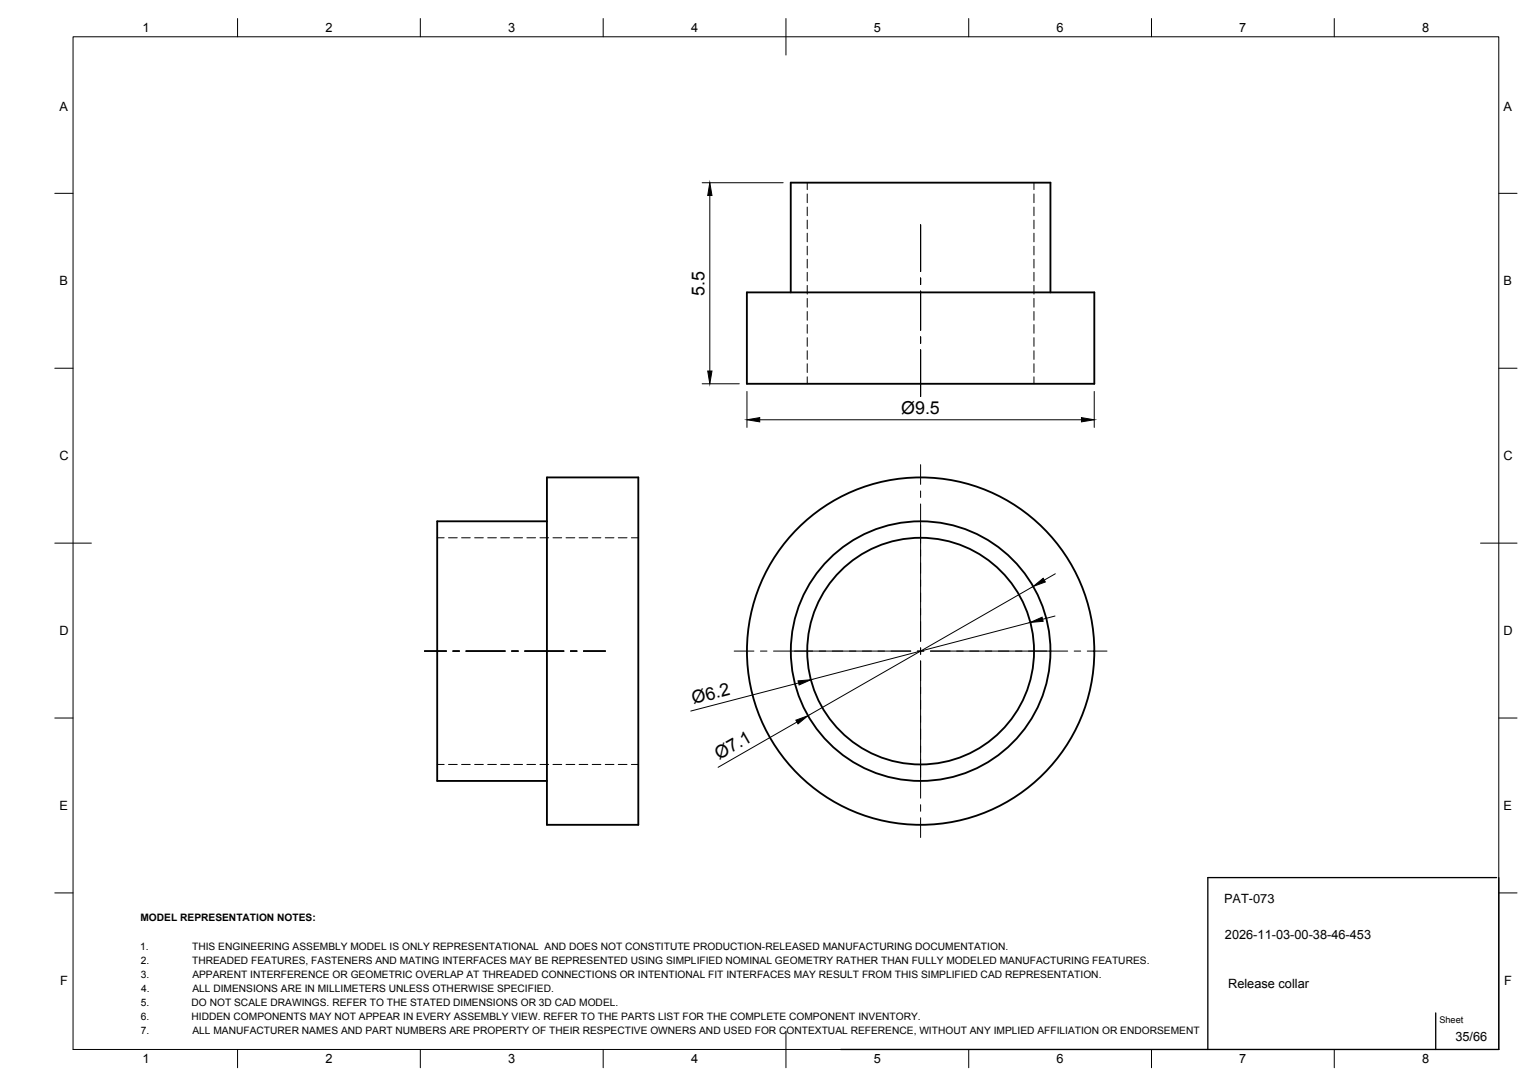
ISO-10303-21;
HEADER;
/* Generated by software containing ST-Developer
 * from STEP Tools, Inc. (www.steptools.com) 
 */

FILE_DESCRIPTION(
/* description */ ('Manual piston pump'),
/* implementation_level */ '2;1');

FILE_NAME(
/* name */ 'Release collar.step',
/* time_stamp */ '2026-11-02T16:54:23-08:00',
/* author */ (''),
/* organization */ (''),
/* preprocessor_version */ 'ST-DEVELOPER v20.2',
/* originating_system */ 'Autodesk Translation Framework v15.17.0.0',
/* authorisation */ '');

FILE_SCHEMA (('AUTOMOTIVE_DESIGN { 1 0 10303 214 3 1 1 }'));
ENDSEC;

DATA;
#10=MECHANICAL_DESIGN_GEOMETRIC_PRESENTATION_REPRESENTATION('',(#729),#19043);
#595=SHAPE_REPRESENTATION_RELATIONSHIP('SRR','None',#19343,#658);
#658=ADVANCED_BREP_SHAPE_REPRESENTATION('',(#799),#19010);
#729=STYLED_ITEM('',(#19661),#799);
#799=MANIFOLD_SOLID_BREP('Body1',#9515);
#990=FACE_BOUND('',#2393,.T.);
#991=FACE_BOUND('',#2396,.T.);
#992=FACE_BOUND('',#2399,.T.);
#1227=CYLINDRICAL_SURFACE('',#10992,0.475);
#1228=CYLINDRICAL_SURFACE('',#10996,0.355);
#1229=CYLINDRICAL_SURFACE('',#11000,0.31);
#1654=FACE_OUTER_BOUND('',#2392,.T.);
#1655=FACE_OUTER_BOUND('',#2394,.T.);
#1656=FACE_OUTER_BOUND('',#2395,.T.);
#1657=FACE_OUTER_BOUND('',#2397,.T.);
#1658=FACE_OUTER_BOUND('',#2398,.T.);
#1659=FACE_OUTER_BOUND('',#2400,.T.);
#2392=EDGE_LOOP('',(#7773));
#2393=EDGE_LOOP('',(#7774));
#2394=EDGE_LOOP('',(#7775,#7776,#7777,#7778));
#2395=EDGE_LOOP('',(#7779));
#2396=EDGE_LOOP('',(#7780));
#2397=EDGE_LOOP('',(#7781,#7782,#7783,#7784));
#2398=EDGE_LOOP('',(#7785));
#2399=EDGE_LOOP('',(#7786));
#2400=EDGE_LOOP('',(#7787,#7788,#7789,#7790));
#2998=CIRCLE('',#10990,0.475);
#2999=CIRCLE('',#10991,0.31);
#3000=CIRCLE('',#10993,0.475);
#3001=CIRCLE('',#10995,0.355);
#3002=CIRCLE('',#10997,0.355);
#3003=CIRCLE('',#10999,0.31);
#3517=LINE('',#17256,#4121);
#3518=LINE('',#17263,#4122);
#3519=LINE('',#17268,#4123);
#4121=VECTOR('',#13367,0.475);
#4122=VECTOR('',#13376,0.355);
#4123=VECTOR('',#13383,0.31);
#4860=VERTEX_POINT('',#17249);
#4861=VERTEX_POINT('',#17251);
#4862=VERTEX_POINT('',#17254);
#4863=VERTEX_POINT('',#17258);
#4864=VERTEX_POINT('',#17261);
#4865=VERTEX_POINT('',#17265);
#5873=EDGE_CURVE('',#4860,#4860,#2998,.T.);
#5874=EDGE_CURVE('',#4861,#4861,#2999,.T.);
#5875=EDGE_CURVE('',#4862,#4862,#3000,.T.);
#5876=EDGE_CURVE('',#4862,#4860,#3517,.T.);
#5877=EDGE_CURVE('',#4863,#4863,#3001,.T.);
#5878=EDGE_CURVE('',#4864,#4864,#3002,.T.);
#5879=EDGE_CURVE('',#4864,#4863,#3518,.T.);
#5880=EDGE_CURVE('',#4865,#4865,#3003,.T.);
#5881=EDGE_CURVE('',#4865,#4861,#3519,.T.);
#7773=ORIENTED_EDGE('',*,*,#5873,.F.);
#7774=ORIENTED_EDGE('',*,*,#5874,.T.);
#7775=ORIENTED_EDGE('',*,*,#5875,.F.);
#7776=ORIENTED_EDGE('',*,*,#5876,.T.);
#7777=ORIENTED_EDGE('',*,*,#5873,.T.);
#7778=ORIENTED_EDGE('',*,*,#5876,.F.);
#7779=ORIENTED_EDGE('',*,*,#5875,.T.);
#7780=ORIENTED_EDGE('',*,*,#5877,.F.);
#7781=ORIENTED_EDGE('',*,*,#5878,.F.);
#7782=ORIENTED_EDGE('',*,*,#5879,.T.);
#7783=ORIENTED_EDGE('',*,*,#5877,.T.);
#7784=ORIENTED_EDGE('',*,*,#5879,.F.);
#7785=ORIENTED_EDGE('',*,*,#5878,.T.);
#7786=ORIENTED_EDGE('',*,*,#5880,.F.);
#7787=ORIENTED_EDGE('',*,*,#5880,.T.);
#7788=ORIENTED_EDGE('',*,*,#5881,.T.);
#7789=ORIENTED_EDGE('',*,*,#5874,.F.);
#7790=ORIENTED_EDGE('',*,*,#5881,.F.);
#8764=PLANE('',#10989);
#8765=PLANE('',#10994);
#8766=PLANE('',#10998);
#9259=ADVANCED_FACE('',(#1654,#990),#8764,.T.);
#9260=ADVANCED_FACE('',(#1655),#1227,.T.);
#9261=ADVANCED_FACE('',(#1656,#991),#8765,.T.);
#9262=ADVANCED_FACE('',(#1657),#1228,.T.);
#9263=ADVANCED_FACE('',(#1658,#992),#8766,.T.);
#9264=ADVANCED_FACE('',(#1659),#1229,.F.);
#9515=CLOSED_SHELL('',(#9259,#9260,#9261,#9262,#9263,#9264));
#10988=AXIS2_PLACEMENT_3D('',#17247,#13355,#13356);
#10989=AXIS2_PLACEMENT_3D('',#17248,#13357,#13358);
#10990=AXIS2_PLACEMENT_3D('',#17250,#13359,#13360);
#10991=AXIS2_PLACEMENT_3D('',#17252,#13361,#13362);
#10992=AXIS2_PLACEMENT_3D('',#17253,#13363,#13364);
#10993=AXIS2_PLACEMENT_3D('',#17255,#13365,#13366);
#10994=AXIS2_PLACEMENT_3D('',#17257,#13368,#13369);
#10995=AXIS2_PLACEMENT_3D('',#17259,#13370,#13371);
#10996=AXIS2_PLACEMENT_3D('',#17260,#13372,#13373);
#10997=AXIS2_PLACEMENT_3D('',#17262,#13374,#13375);
#10998=AXIS2_PLACEMENT_3D('',#17264,#13377,#13378);
#10999=AXIS2_PLACEMENT_3D('',#17266,#13379,#13380);
#11000=AXIS2_PLACEMENT_3D('',#17267,#13381,#13382);
#13355=DIRECTION('axis',(0.,0.,1.));
#13356=DIRECTION('refdir',(1.,0.,0.));
#13357=DIRECTION('center_axis',(0.,1.,0.));
#13358=DIRECTION('ref_axis',(0.,0.,1.));
#13359=DIRECTION('center_axis',(0.,-1.,0.));
#13360=DIRECTION('ref_axis',(1.,0.,0.));
#13361=DIRECTION('center_axis',(0.,-1.,0.));
#13362=DIRECTION('ref_axis',(1.,0.,0.));
#13363=DIRECTION('center_axis',(0.,-1.,0.));
#13364=DIRECTION('ref_axis',(1.,0.,0.));
#13365=DIRECTION('center_axis',(0.,-1.,0.));
#13366=DIRECTION('ref_axis',(1.,0.,0.));
#13367=DIRECTION('',(0.,1.,0.));
#13368=DIRECTION('center_axis',(0.,-1.,0.));
#13369=DIRECTION('ref_axis',(0.,0.,-1.));
#13370=DIRECTION('center_axis',(0.,-1.,0.));
#13371=DIRECTION('ref_axis',(1.,0.,0.));
#13372=DIRECTION('center_axis',(0.,-1.,0.));
#13373=DIRECTION('ref_axis',(1.,0.,0.));
#13374=DIRECTION('center_axis',(0.,-1.,0.));
#13375=DIRECTION('ref_axis',(1.,0.,0.));
#13376=DIRECTION('',(0.,1.,0.));
#13377=DIRECTION('center_axis',(0.,-1.,0.));
#13378=DIRECTION('ref_axis',(0.,0.,-1.));
#13379=DIRECTION('center_axis',(0.,-1.,0.));
#13380=DIRECTION('ref_axis',(1.,0.,0.));
#13381=DIRECTION('center_axis',(0.,-1.,0.));
#13382=DIRECTION('ref_axis',(1.,0.,0.));
#13383=DIRECTION('',(0.,1.,0.));
#17247=CARTESIAN_POINT('',(0.,0.,0.));
#17248=CARTESIAN_POINT('Origin',(0.475,1.95,0.));
#17249=CARTESIAN_POINT('',(-0.475,1.95,-5.81707229594993E-17));
#17250=CARTESIAN_POINT('Origin',(0.,1.95,0.));
#17251=CARTESIAN_POINT('',(-0.31,1.95,-3.7964050773568E-17));
#17252=CARTESIAN_POINT('Origin',(0.,1.95,0.));
#17253=CARTESIAN_POINT('Origin',(0.,1.825,0.));
#17254=CARTESIAN_POINT('',(-0.475,1.7,-5.81707229594993E-17));
#17255=CARTESIAN_POINT('Origin',(0.,1.7,0.));
#17256=CARTESIAN_POINT('',(-0.475,1.825,-5.81707229594993E-17));
#17257=CARTESIAN_POINT('Origin',(0.355,1.7,0.));
#17258=CARTESIAN_POINT('',(-0.355,1.7,-4.3474961369731E-17));
#17259=CARTESIAN_POINT('Origin',(0.,1.7,0.));
#17260=CARTESIAN_POINT('Origin',(0.,1.55,0.));
#17261=CARTESIAN_POINT('',(-0.355,1.4,-4.3474961369731E-17));
#17262=CARTESIAN_POINT('Origin',(0.,1.4,0.));
#17263=CARTESIAN_POINT('',(-0.355,1.55,-4.3474961369731E-17));
#17264=CARTESIAN_POINT('Origin',(0.31,1.4,0.));
#17265=CARTESIAN_POINT('',(-0.31,1.4,-3.7964050773568E-17));
#17266=CARTESIAN_POINT('Origin',(0.,1.4,0.));
#17267=CARTESIAN_POINT('Origin',(0.,1.675,0.));
#17268=CARTESIAN_POINT('',(-0.31,1.675,-3.7964050773568E-17));
#18939=UNCERTAINTY_MEASURE_WITH_UNIT(LENGTH_MEASURE(0.001),#19044,
'DISTANCE_ACCURACY_VALUE',
'Maximum model space distance between geometric entities at asserted c
onnectivities');
#18972=UNCERTAINTY_MEASURE_WITH_UNIT(LENGTH_MEASURE(0.001),#19044,
'DISTANCE_ACCURACY_VALUE',
'Maximum model space distance between geometric entities at asserted c
onnectivities');
#19010=(
GEOMETRIC_REPRESENTATION_CONTEXT(3)
GLOBAL_UNCERTAINTY_ASSIGNED_CONTEXT((#18939))
GLOBAL_UNIT_ASSIGNED_CONTEXT((#19044,#19046,#19047))
REPRESENTATION_CONTEXT('','3D')
);
#19043=(
GEOMETRIC_REPRESENTATION_CONTEXT(3)
GLOBAL_UNCERTAINTY_ASSIGNED_CONTEXT((#18972))
GLOBAL_UNIT_ASSIGNED_CONTEXT((#19044,#19046,#19047))
REPRESENTATION_CONTEXT('','3D')
);
#19044=(
LENGTH_UNIT()
NAMED_UNIT(*)
SI_UNIT(.CENTI.,.METRE.)
);
#19046=(
NAMED_UNIT(*)
PLANE_ANGLE_UNIT()
SI_UNIT($,.RADIAN.)
);
#19047=(
NAMED_UNIT(*)
SI_UNIT($,.STERADIAN.)
SOLID_ANGLE_UNIT()
);
#19085=SHAPE_DEFINITION_REPRESENTATION(#19160,#19343);
#19160=PRODUCT_DEFINITION_SHAPE('',$,#19414);
#19343=SHAPE_REPRESENTATION('',(#10988),#19010);
#19376=PRODUCT_DEFINITION_CONTEXT('part definition',#19588,'design');
#19414=PRODUCT_DEFINITION('2026-11-03-00-38-46-453','Release collar',#19484,
#19376);
#19484=PRODUCT_DEFINITION_FORMATION('',$,#19627);
#19588=APPLICATION_CONTEXT(
'Core Data for Automotive Mechanical Design Process');
#19589=PRODUCT_CONTEXT('part definition',#19588,'mechanical');
#19627=PRODUCT('2026-11-03-00-38-46-453','Release collar',
'Release collar',(#19589));
#19661=PRESENTATION_STYLE_ASSIGNMENT((#19667));
#19667=SURFACE_STYLE_USAGE(.BOTH.,#19673);
#19673=SURFACE_SIDE_STYLE('',(#19679));
#19679=SURFACE_STYLE_FILL_AREA(#19685);
#19685=FILL_AREA_STYLE('CAD Library Painted - Engineering blue',(#19691));
#19691=FILL_AREA_STYLE_COLOUR('CAD Library Painted - Engineering blue',
#19697);
#19697=COLOUR_RGB('CAD Library Painted - Engineering blue',0.12156862745098,
0.356862745098039,0.6);
ENDSEC;
END-ISO-10303-21;
